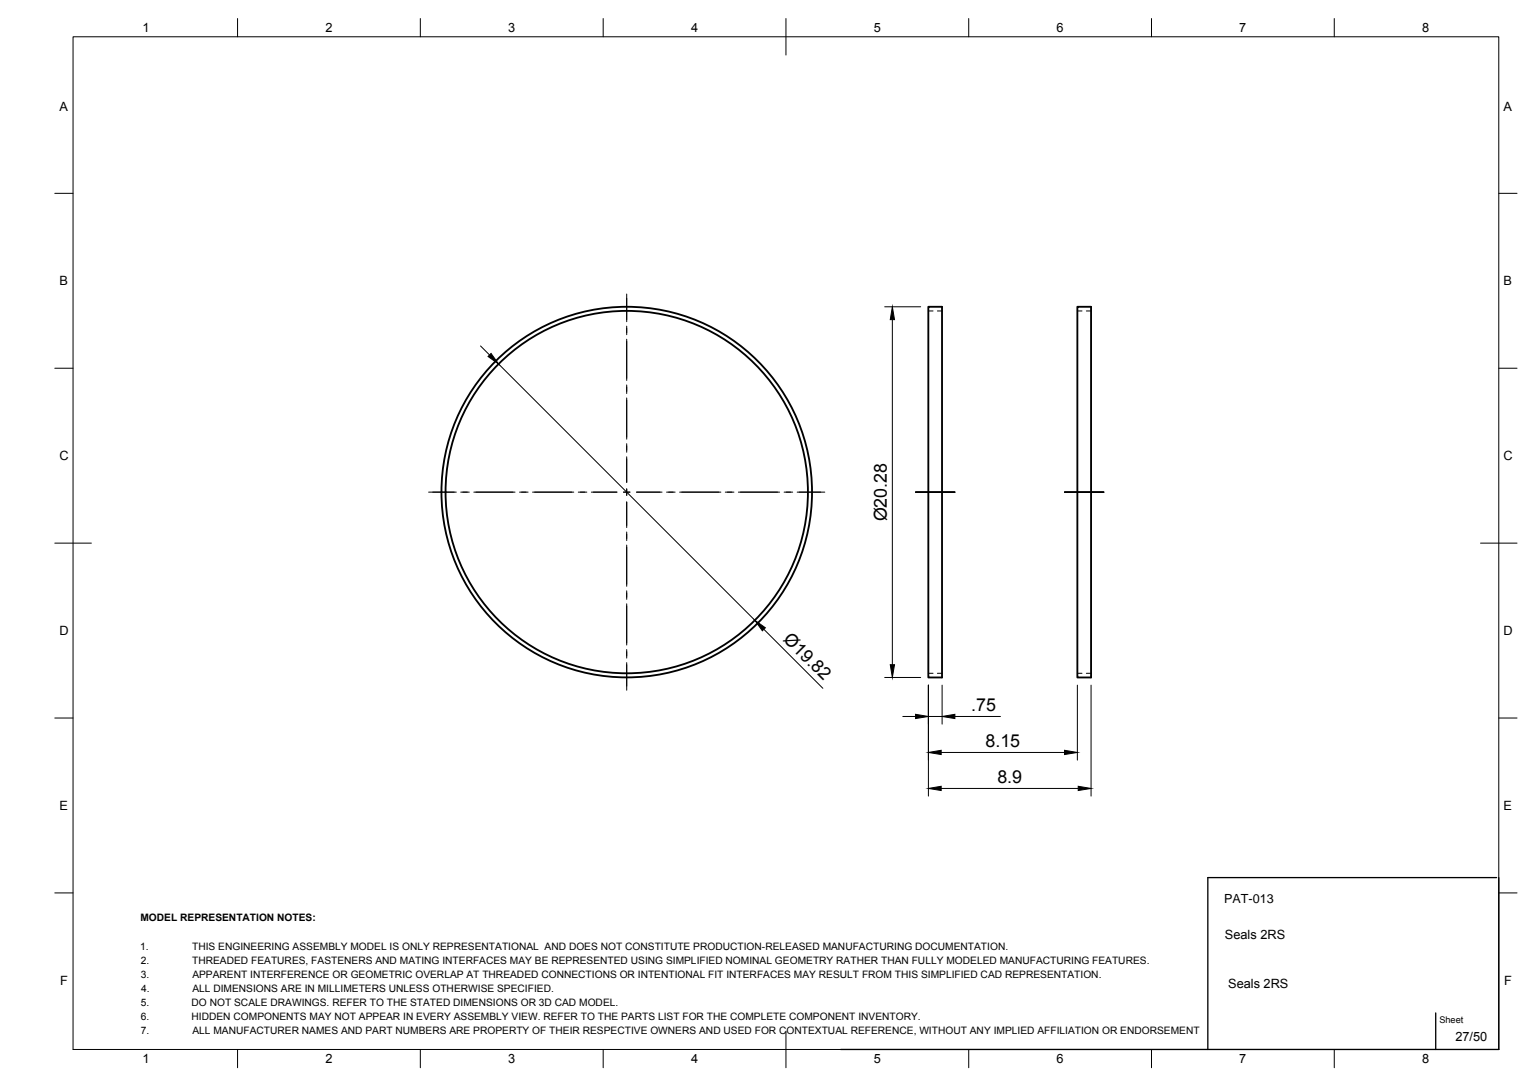
ISO-10303-21;
HEADER;
/* Generated by software containing ST-Developer
 * from STEP Tools, Inc. (www.steptools.com) 
 */

FILE_DESCRIPTION(
/* description */ ('Belt-driven linear axis on 2020 extrusion'),
/* implementation_level */ '2;1');

FILE_NAME(
/* name */ 'Seals 2RS.step',
/* time_stamp */ '2026-10-28T03:26:09-07:00',
/* author */ (''),
/* organization */ (''),
/* preprocessor_version */ 'ST-DEVELOPER v20.2',
/* originating_system */ 'Autodesk Translation Framework v15.17.0.0',
/* authorisation */ '');

FILE_SCHEMA (('AUTOMOTIVE_DESIGN { 1 0 10303 214 3 1 1 }'));
ENDSEC;

DATA;
#10=MECHANICAL_DESIGN_GEOMETRIC_PRESENTATION_REPRESENTATION('',(#637,#638),#20096);
#536=SHAPE_REPRESENTATION_RELATIONSHIP('SRR','None',#20333,#582);
#582=ADVANCED_BREP_SHAPE_REPRESENTATION('',(#693,#694),#20064);
#637=STYLED_ITEM('',(#20650),#693);
#638=STYLED_ITEM('',(#20650),#694);
#693=MANIFOLD_SOLID_BREP('Body1',#10950);
#694=MANIFOLD_SOLID_BREP('Body2',#10951);
#809=FACE_BOUND('',#2221,.T.);
#810=FACE_BOUND('',#2224,.T.);
#811=FACE_BOUND('',#2227,.T.);
#812=FACE_BOUND('',#2230,.T.);
#1018=PLANE('',#12029);
#1019=PLANE('',#12034);
#1020=PLANE('',#12037);
#1021=PLANE('',#12042);
#1507=FACE_OUTER_BOUND('',#2220,.T.);
#1508=FACE_OUTER_BOUND('',#2222,.T.);
#1509=FACE_OUTER_BOUND('',#2223,.T.);
#1510=FACE_OUTER_BOUND('',#2225,.T.);
#1511=FACE_OUTER_BOUND('',#2226,.T.);
#1512=FACE_OUTER_BOUND('',#2228,.T.);
#1513=FACE_OUTER_BOUND('',#2229,.T.);
#1514=FACE_OUTER_BOUND('',#2231,.T.);
#2220=EDGE_LOOP('',(#8413));
#2221=EDGE_LOOP('',(#8414));
#2222=EDGE_LOOP('',(#8415,#8416,#8417,#8418));
#2223=EDGE_LOOP('',(#8419));
#2224=EDGE_LOOP('',(#8420));
#2225=EDGE_LOOP('',(#8421,#8422,#8423,#8424));
#2226=EDGE_LOOP('',(#8425));
#2227=EDGE_LOOP('',(#8426));
#2228=EDGE_LOOP('',(#8427,#8428,#8429,#8430));
#2229=EDGE_LOOP('',(#8431));
#2230=EDGE_LOOP('',(#8432));
#2231=EDGE_LOOP('',(#8433,#8434,#8435,#8436));
#2967=LINE('',#17833,#3824);
#2968=LINE('',#17838,#3825);
#2969=LINE('',#17847,#3826);
#2970=LINE('',#17852,#3827);
#3824=VECTOR('',#14175,1.013815);
#3825=VECTOR('',#14182,0.991185);
#3826=VECTOR('',#14193,1.013815);
#3827=VECTOR('',#14200,0.991185);
#4639=CIRCLE('',#12030,1.013815);
#4640=CIRCLE('',#12031,0.991185);
#4641=CIRCLE('',#12033,1.013815);
#4642=CIRCLE('',#12035,0.991185);
#4643=CIRCLE('',#12038,1.013815);
#4644=CIRCLE('',#12039,0.991185);
#4645=CIRCLE('',#12041,1.013815);
#4646=CIRCLE('',#12043,0.991185);
#5288=VERTEX_POINT('',#17826);
#5289=VERTEX_POINT('',#17828);
#5290=VERTEX_POINT('',#17831);
#5291=VERTEX_POINT('',#17835);
#5292=VERTEX_POINT('',#17840);
#5293=VERTEX_POINT('',#17842);
#5294=VERTEX_POINT('',#17845);
#5295=VERTEX_POINT('',#17849);
#6421=EDGE_CURVE('',#5288,#5288,#4639,.T.);
#6422=EDGE_CURVE('',#5289,#5289,#4640,.T.);
#6423=EDGE_CURVE('',#5290,#5290,#4641,.T.);
#6424=EDGE_CURVE('',#5290,#5288,#2967,.T.);
#6425=EDGE_CURVE('',#5291,#5291,#4642,.T.);
#6426=EDGE_CURVE('',#5291,#5289,#2968,.T.);
#6427=EDGE_CURVE('',#5292,#5292,#4643,.T.);
#6428=EDGE_CURVE('',#5293,#5293,#4644,.T.);
#6429=EDGE_CURVE('',#5294,#5294,#4645,.T.);
#6430=EDGE_CURVE('',#5294,#5292,#2969,.T.);
#6431=EDGE_CURVE('',#5295,#5295,#4646,.T.);
#6432=EDGE_CURVE('',#5295,#5293,#2970,.T.);
#8413=ORIENTED_EDGE('',*,*,#6421,.F.);
#8414=ORIENTED_EDGE('',*,*,#6422,.T.);
#8415=ORIENTED_EDGE('',*,*,#6423,.F.);
#8416=ORIENTED_EDGE('',*,*,#6424,.T.);
#8417=ORIENTED_EDGE('',*,*,#6421,.T.);
#8418=ORIENTED_EDGE('',*,*,#6424,.F.);
#8419=ORIENTED_EDGE('',*,*,#6423,.T.);
#8420=ORIENTED_EDGE('',*,*,#6425,.F.);
#8421=ORIENTED_EDGE('',*,*,#6425,.T.);
#8422=ORIENTED_EDGE('',*,*,#6426,.T.);
#8423=ORIENTED_EDGE('',*,*,#6422,.F.);
#8424=ORIENTED_EDGE('',*,*,#6426,.F.);
#8425=ORIENTED_EDGE('',*,*,#6427,.F.);
#8426=ORIENTED_EDGE('',*,*,#6428,.T.);
#8427=ORIENTED_EDGE('',*,*,#6429,.F.);
#8428=ORIENTED_EDGE('',*,*,#6430,.T.);
#8429=ORIENTED_EDGE('',*,*,#6427,.T.);
#8430=ORIENTED_EDGE('',*,*,#6430,.F.);
#8431=ORIENTED_EDGE('',*,*,#6429,.T.);
#8432=ORIENTED_EDGE('',*,*,#6431,.F.);
#8433=ORIENTED_EDGE('',*,*,#6431,.T.);
#8434=ORIENTED_EDGE('',*,*,#6432,.T.);
#8435=ORIENTED_EDGE('',*,*,#6428,.F.);
#8436=ORIENTED_EDGE('',*,*,#6432,.F.);
#10183=CYLINDRICAL_SURFACE('',#12032,1.013815);
#10184=CYLINDRICAL_SURFACE('',#12036,0.991185);
#10185=CYLINDRICAL_SURFACE('',#12040,1.013815);
#10186=CYLINDRICAL_SURFACE('',#12044,0.991185);
#10558=ADVANCED_FACE('',(#1507,#809),#1018,.T.);
#10559=ADVANCED_FACE('',(#1508),#10183,.T.);
#10560=ADVANCED_FACE('',(#1509,#810),#1019,.T.);
#10561=ADVANCED_FACE('',(#1510),#10184,.F.);
#10562=ADVANCED_FACE('',(#1511,#811),#1020,.T.);
#10563=ADVANCED_FACE('',(#1512),#10185,.T.);
#10564=ADVANCED_FACE('',(#1513,#812),#1021,.T.);
#10565=ADVANCED_FACE('',(#1514),#10186,.F.);
#10950=CLOSED_SHELL('',(#10558,#10559,#10560,#10561));
#10951=CLOSED_SHELL('',(#10562,#10563,#10564,#10565));
#12028=AXIS2_PLACEMENT_3D('',#17824,#14163,#14164);
#12029=AXIS2_PLACEMENT_3D('',#17825,#14165,#14166);
#12030=AXIS2_PLACEMENT_3D('',#17827,#14167,#14168);
#12031=AXIS2_PLACEMENT_3D('',#17829,#14169,#14170);
#12032=AXIS2_PLACEMENT_3D('',#17830,#14171,#14172);
#12033=AXIS2_PLACEMENT_3D('',#17832,#14173,#14174);
#12034=AXIS2_PLACEMENT_3D('',#17834,#14176,#14177);
#12035=AXIS2_PLACEMENT_3D('',#17836,#14178,#14179);
#12036=AXIS2_PLACEMENT_3D('',#17837,#14180,#14181);
#12037=AXIS2_PLACEMENT_3D('',#17839,#14183,#14184);
#12038=AXIS2_PLACEMENT_3D('',#17841,#14185,#14186);
#12039=AXIS2_PLACEMENT_3D('',#17843,#14187,#14188);
#12040=AXIS2_PLACEMENT_3D('',#17844,#14189,#14190);
#12041=AXIS2_PLACEMENT_3D('',#17846,#14191,#14192);
#12042=AXIS2_PLACEMENT_3D('',#17848,#14194,#14195);
#12043=AXIS2_PLACEMENT_3D('',#17850,#14196,#14197);
#12044=AXIS2_PLACEMENT_3D('',#17851,#14198,#14199);
#14163=DIRECTION('axis',(0.,0.,1.));
#14164=DIRECTION('refdir',(1.,0.,0.));
#14165=DIRECTION('center_axis',(0.,1.,0.));
#14166=DIRECTION('ref_axis',(0.,0.,1.));
#14167=DIRECTION('center_axis',(0.,-1.,0.));
#14168=DIRECTION('ref_axis',(1.,0.,0.));
#14169=DIRECTION('center_axis',(0.,-1.,0.));
#14170=DIRECTION('ref_axis',(1.,0.,0.));
#14171=DIRECTION('center_axis',(0.,-1.,0.));
#14172=DIRECTION('ref_axis',(1.,0.,0.));
#14173=DIRECTION('center_axis',(0.,-1.,0.));
#14174=DIRECTION('ref_axis',(1.,0.,0.));
#14175=DIRECTION('',(0.,1.,0.));
#14176=DIRECTION('center_axis',(0.,-1.,0.));
#14177=DIRECTION('ref_axis',(0.,0.,-1.));
#14178=DIRECTION('center_axis',(0.,-1.,0.));
#14179=DIRECTION('ref_axis',(1.,0.,0.));
#14180=DIRECTION('center_axis',(0.,-1.,0.));
#14181=DIRECTION('ref_axis',(1.,0.,0.));
#14182=DIRECTION('',(0.,1.,0.));
#14183=DIRECTION('center_axis',(0.,1.,0.));
#14184=DIRECTION('ref_axis',(0.,0.,1.));
#14185=DIRECTION('center_axis',(0.,-1.,0.));
#14186=DIRECTION('ref_axis',(1.,0.,0.));
#14187=DIRECTION('center_axis',(0.,-1.,0.));
#14188=DIRECTION('ref_axis',(1.,0.,0.));
#14189=DIRECTION('center_axis',(0.,-1.,0.));
#14190=DIRECTION('ref_axis',(1.,0.,0.));
#14191=DIRECTION('center_axis',(0.,-1.,0.));
#14192=DIRECTION('ref_axis',(1.,0.,0.));
#14193=DIRECTION('',(0.,1.,0.));
#14194=DIRECTION('center_axis',(0.,-1.,0.));
#14195=DIRECTION('ref_axis',(0.,0.,-1.));
#14196=DIRECTION('center_axis',(0.,-1.,0.));
#14197=DIRECTION('ref_axis',(1.,0.,0.));
#14198=DIRECTION('center_axis',(0.,-1.,0.));
#14199=DIRECTION('ref_axis',(1.,0.,0.));
#14200=DIRECTION('',(0.,1.,0.));
#17824=CARTESIAN_POINT('',(0.,0.,0.));
#17825=CARTESIAN_POINT('Origin',(1.013815,0.445,0.));
#17826=CARTESIAN_POINT('',(-1.013815,0.445,-1.24156529467757E-16));
#17827=CARTESIAN_POINT('Origin',(0.,0.445,0.));
#17828=CARTESIAN_POINT('',(-0.991185,0.445,-1.21385153761287E-16));
#17829=CARTESIAN_POINT('Origin',(0.,0.445,0.));
#17830=CARTESIAN_POINT('Origin',(0.,0.4075,0.));
#17831=CARTESIAN_POINT('',(-1.013815,0.37,-1.24156529467757E-16));
#17832=CARTESIAN_POINT('Origin',(0.,0.37,0.));
#17833=CARTESIAN_POINT('',(-1.013815,0.4075,-1.24156529467757E-16));
#17834=CARTESIAN_POINT('Origin',(0.991185,0.37,0.));
#17835=CARTESIAN_POINT('',(-0.991185,0.37,-1.21385153761287E-16));
#17836=CARTESIAN_POINT('Origin',(0.,0.37,0.));
#17837=CARTESIAN_POINT('Origin',(0.,0.4075,0.));
#17838=CARTESIAN_POINT('',(-0.991185,0.4075,-1.21385153761287E-16));
#17839=CARTESIAN_POINT('Origin',(1.013815,-0.37,0.));
#17840=CARTESIAN_POINT('',(-1.013815,-0.37,-1.24156529467757E-16));
#17841=CARTESIAN_POINT('Origin',(0.,-0.37,0.));
#17842=CARTESIAN_POINT('',(-0.991185,-0.37,-1.21385153761287E-16));
#17843=CARTESIAN_POINT('Origin',(0.,-0.37,0.));
#17844=CARTESIAN_POINT('Origin',(0.,-0.4075,0.));
#17845=CARTESIAN_POINT('',(-1.013815,-0.445,-1.24156529467757E-16));
#17846=CARTESIAN_POINT('Origin',(0.,-0.445,0.));
#17847=CARTESIAN_POINT('',(-1.013815,-0.4075,-1.24156529467757E-16));
#17848=CARTESIAN_POINT('Origin',(0.991185,-0.445,0.));
#17849=CARTESIAN_POINT('',(-0.991185,-0.445,-1.21385153761287E-16));
#17850=CARTESIAN_POINT('Origin',(0.,-0.445,0.));
#17851=CARTESIAN_POINT('Origin',(0.,-0.4075,0.));
#17852=CARTESIAN_POINT('',(-0.991185,-0.4075,-1.21385153761287E-16));
#20010=UNCERTAINTY_MEASURE_WITH_UNIT(LENGTH_MEASURE(0.001),#20097,
'DISTANCE_ACCURACY_VALUE',
'Maximum model space distance between geometric entities at asserted c
onnectivities');
#20042=UNCERTAINTY_MEASURE_WITH_UNIT(LENGTH_MEASURE(0.001),#20097,
'DISTANCE_ACCURACY_VALUE',
'Maximum model space distance between geometric entities at asserted c
onnectivities');
#20064=(
GEOMETRIC_REPRESENTATION_CONTEXT(3)
GLOBAL_UNCERTAINTY_ASSIGNED_CONTEXT((#20010))
GLOBAL_UNIT_ASSIGNED_CONTEXT((#20097,#20099,#20100))
REPRESENTATION_CONTEXT('','3D')
);
#20096=(
GEOMETRIC_REPRESENTATION_CONTEXT(3)
GLOBAL_UNCERTAINTY_ASSIGNED_CONTEXT((#20042))
GLOBAL_UNIT_ASSIGNED_CONTEXT((#20097,#20099,#20100))
REPRESENTATION_CONTEXT('','3D')
);
#20097=(
LENGTH_UNIT()
NAMED_UNIT(*)
SI_UNIT(.CENTI.,.METRE.)
);
#20099=(
NAMED_UNIT(*)
PLANE_ANGLE_UNIT()
SI_UNIT($,.RADIAN.)
);
#20100=(
NAMED_UNIT(*)
SI_UNIT($,.STERADIAN.)
SOLID_ANGLE_UNIT()
);
#20122=SHAPE_DEFINITION_REPRESENTATION(#20175,#20333);
#20175=PRODUCT_DEFINITION_SHAPE('',$,#20387);
#20333=SHAPE_REPRESENTATION('',(#12028),#20064);
#20365=PRODUCT_DEFINITION_CONTEXT('part definition',#20526,'design');
#20387=PRODUCT_DEFINITION('Seals 2RS','Seals 2RS',#20440,#20365);
#20440=PRODUCT_DEFINITION_FORMATION('',$,#20549);
#20526=APPLICATION_CONTEXT(
'Core Data for Automotive Mechanical Design Process');
#20527=PRODUCT_CONTEXT('part definition',#20526,'mechanical');
#20549=PRODUCT('Seals 2RS','Seals 2RS','Seals 2RS',(#20527));
#20644=COLOUR_RGB('Grey',0.48,0.52,0.57);
#20645=FILL_AREA_STYLE_COLOUR('',#20644);
#20646=FILL_AREA_STYLE('',(#20645));
#20647=SURFACE_STYLE_FILL_AREA(#20646);
#20648=SURFACE_SIDE_STYLE('',(#20647));
#20649=SURFACE_STYLE_USAGE(.BOTH.,#20648);
#20650=PRESENTATION_STYLE_ASSIGNMENT((#20649));
ENDSEC;
END-ISO-10303-21;
